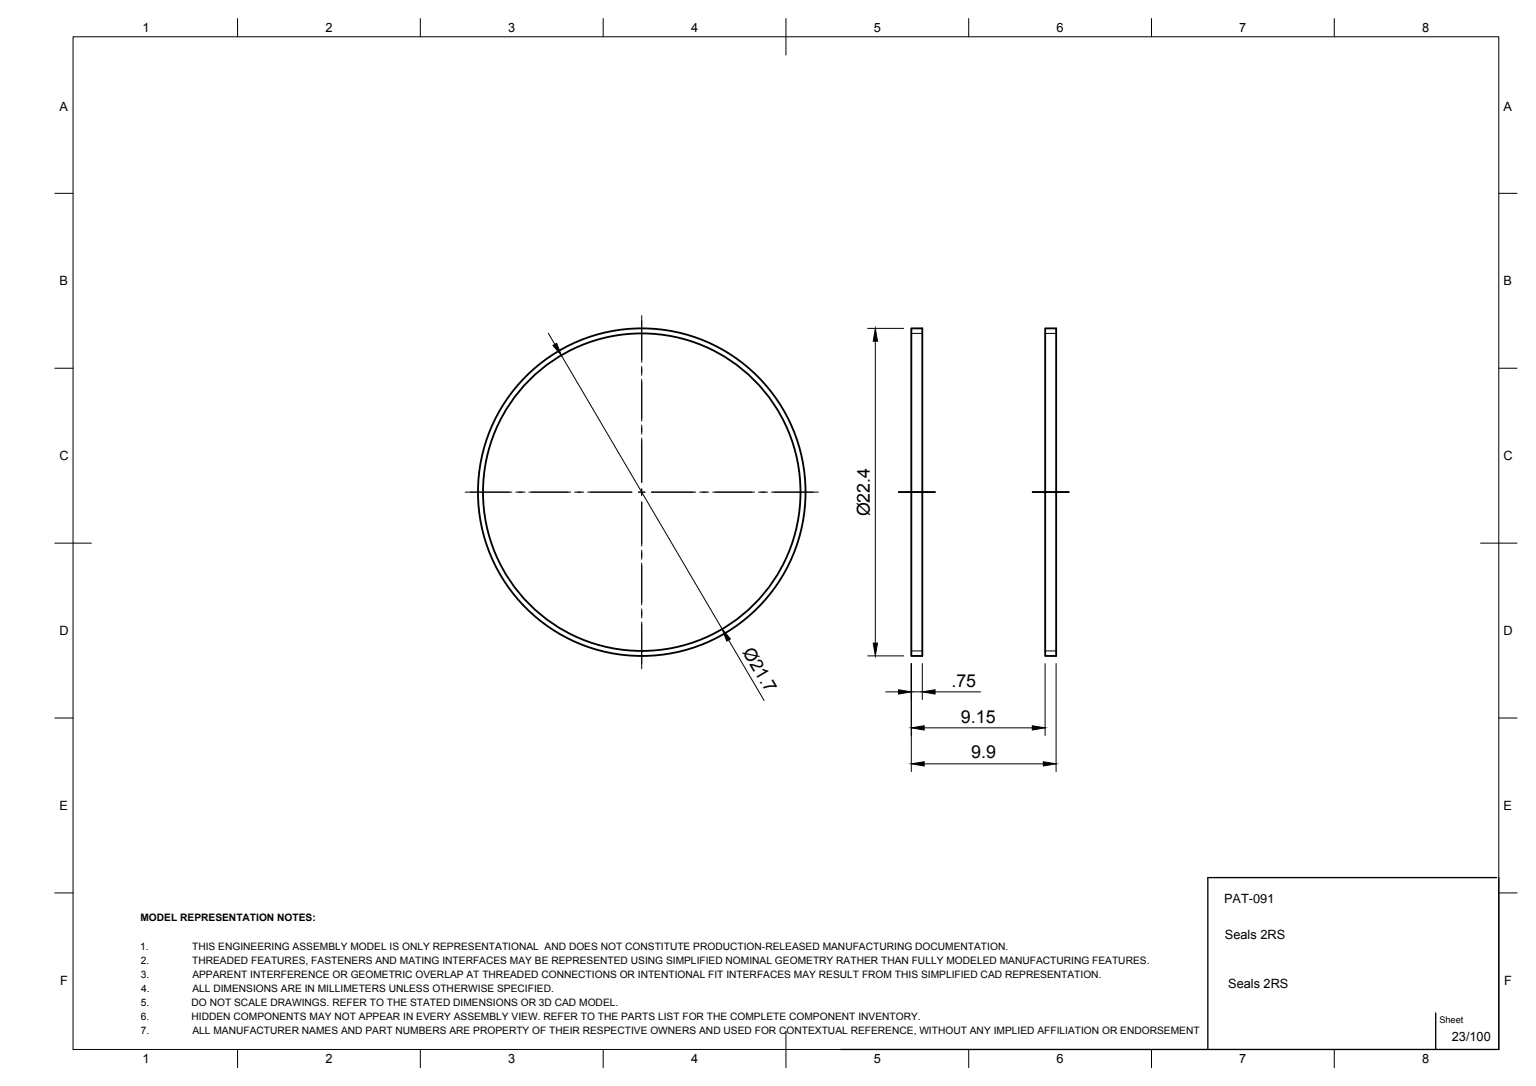
ISO-10303-21;
HEADER;
/* Generated by software containing ST-Developer
 * from STEP Tools, Inc. (www.steptools.com) 
 */

FILE_DESCRIPTION(
/* description */ ('PAT-091'),
/* implementation_level */ '2;1');

FILE_NAME(
/* name */ 'Seals 2RS.step',
/* time_stamp */ '2026-10-27T15:34:44-07:00',
/* author */ (''),
/* organization */ (''),
/* preprocessor_version */ 'ST-DEVELOPER v20.2',
/* originating_system */ 'Autodesk Translation Framework v15.17.0.0',
/* authorisation */ '');

FILE_SCHEMA (('AUTOMOTIVE_DESIGN { 1 0 10303 214 3 1 1 }'));
ENDSEC;

DATA;
#10=MECHANICAL_DESIGN_GEOMETRIC_PRESENTATION_REPRESENTATION('',(#1086,#1087),#25100);
#854=SHAPE_REPRESENTATION_RELATIONSHIP('SRR','None',#25622,#964);
#964=ADVANCED_BREP_SHAPE_REPRESENTATION('',(#1207,#1208),#25092);
#1086=STYLED_ITEM('',(#26191),#1207);
#1087=STYLED_ITEM('',(#26191),#1208);
#1207=MANIFOLD_SOLID_BREP('Body1',#13366);
#1208=MANIFOLD_SOLID_BREP('Body2',#13367);
#1621=FACE_BOUND('',#4065,.T.);
#1622=FACE_BOUND('',#4068,.T.);
#1623=FACE_BOUND('',#4071,.T.);
#1624=FACE_BOUND('',#4074,.T.);
#2042=PLANE('',#16288);
#2043=PLANE('',#16293);
#2044=PLANE('',#16296);
#2045=PLANE('',#16301);
#2840=FACE_OUTER_BOUND('',#4064,.T.);
#2841=FACE_OUTER_BOUND('',#4066,.T.);
#2842=FACE_OUTER_BOUND('',#4067,.T.);
#2843=FACE_OUTER_BOUND('',#4069,.T.);
#2844=FACE_OUTER_BOUND('',#4070,.T.);
#2845=FACE_OUTER_BOUND('',#4072,.T.);
#2846=FACE_OUTER_BOUND('',#4073,.T.);
#2847=FACE_OUTER_BOUND('',#4075,.T.);
#4064=EDGE_LOOP('',(#11954));
#4065=EDGE_LOOP('',(#11955));
#4066=EDGE_LOOP('',(#11956,#11957,#11958,#11959));
#4067=EDGE_LOOP('',(#11960));
#4068=EDGE_LOOP('',(#11961));
#4069=EDGE_LOOP('',(#11962,#11963,#11964,#11965));
#4070=EDGE_LOOP('',(#11966));
#4071=EDGE_LOOP('',(#11967));
#4072=EDGE_LOOP('',(#11968,#11969,#11970,#11971));
#4073=EDGE_LOOP('',(#11972));
#4074=EDGE_LOOP('',(#11973));
#4075=EDGE_LOOP('',(#11974,#11975,#11976,#11977));
#4844=LINE('',#24627,#5584);
#4845=LINE('',#24632,#5585);
#4846=LINE('',#24641,#5586);
#4847=LINE('',#24646,#5587);
#5584=VECTOR('',#20604,1.119765);
#5585=VECTOR('',#20611,1.085235);
#5586=VECTOR('',#20622,1.119765);
#5587=VECTOR('',#20629,1.085235);
#6343=CIRCLE('',#16289,1.119765);
#6344=CIRCLE('',#16290,1.085235);
#6345=CIRCLE('',#16292,1.119765);
#6346=CIRCLE('',#16294,1.085235);
#6347=CIRCLE('',#16297,1.119765);
#6348=CIRCLE('',#16298,1.085235);
#6349=CIRCLE('',#16300,1.119765);
#6350=CIRCLE('',#16302,1.085235);
#7381=VERTEX_POINT('',#24620);
#7382=VERTEX_POINT('',#24622);
#7383=VERTEX_POINT('',#24625);
#7384=VERTEX_POINT('',#24629);
#7385=VERTEX_POINT('',#24634);
#7386=VERTEX_POINT('',#24636);
#7387=VERTEX_POINT('',#24639);
#7388=VERTEX_POINT('',#24643);
#8912=EDGE_CURVE('',#7381,#7381,#6343,.T.);
#8913=EDGE_CURVE('',#7382,#7382,#6344,.T.);
#8914=EDGE_CURVE('',#7383,#7383,#6345,.T.);
#8915=EDGE_CURVE('',#7383,#7381,#4844,.T.);
#8916=EDGE_CURVE('',#7384,#7384,#6346,.T.);
#8917=EDGE_CURVE('',#7384,#7382,#4845,.T.);
#8918=EDGE_CURVE('',#7385,#7385,#6347,.T.);
#8919=EDGE_CURVE('',#7386,#7386,#6348,.T.);
#8920=EDGE_CURVE('',#7387,#7387,#6349,.T.);
#8921=EDGE_CURVE('',#7387,#7385,#4846,.T.);
#8922=EDGE_CURVE('',#7388,#7388,#6350,.T.);
#8923=EDGE_CURVE('',#7388,#7386,#4847,.T.);
#11954=ORIENTED_EDGE('',*,*,#8912,.F.);
#11955=ORIENTED_EDGE('',*,*,#8913,.T.);
#11956=ORIENTED_EDGE('',*,*,#8914,.F.);
#11957=ORIENTED_EDGE('',*,*,#8915,.T.);
#11958=ORIENTED_EDGE('',*,*,#8912,.T.);
#11959=ORIENTED_EDGE('',*,*,#8915,.F.);
#11960=ORIENTED_EDGE('',*,*,#8914,.T.);
#11961=ORIENTED_EDGE('',*,*,#8916,.F.);
#11962=ORIENTED_EDGE('',*,*,#8916,.T.);
#11963=ORIENTED_EDGE('',*,*,#8917,.T.);
#11964=ORIENTED_EDGE('',*,*,#8913,.F.);
#11965=ORIENTED_EDGE('',*,*,#8917,.F.);
#11966=ORIENTED_EDGE('',*,*,#8918,.F.);
#11967=ORIENTED_EDGE('',*,*,#8919,.T.);
#11968=ORIENTED_EDGE('',*,*,#8920,.F.);
#11969=ORIENTED_EDGE('',*,*,#8921,.T.);
#11970=ORIENTED_EDGE('',*,*,#8918,.T.);
#11971=ORIENTED_EDGE('',*,*,#8921,.F.);
#11972=ORIENTED_EDGE('',*,*,#8920,.T.);
#11973=ORIENTED_EDGE('',*,*,#8922,.F.);
#11974=ORIENTED_EDGE('',*,*,#8922,.T.);
#11975=ORIENTED_EDGE('',*,*,#8923,.T.);
#11976=ORIENTED_EDGE('',*,*,#8919,.F.);
#11977=ORIENTED_EDGE('',*,*,#8923,.F.);
#12410=CYLINDRICAL_SURFACE('',#16291,1.119765);
#12411=CYLINDRICAL_SURFACE('',#16295,1.085235);
#12412=CYLINDRICAL_SURFACE('',#16299,1.119765);
#12413=CYLINDRICAL_SURFACE('',#16303,1.085235);
#13207=ADVANCED_FACE('',(#2840,#1621),#2042,.T.);
#13208=ADVANCED_FACE('',(#2841),#12410,.T.);
#13209=ADVANCED_FACE('',(#2842,#1622),#2043,.T.);
#13210=ADVANCED_FACE('',(#2843),#12411,.F.);
#13211=ADVANCED_FACE('',(#2844,#1623),#2044,.T.);
#13212=ADVANCED_FACE('',(#2845),#12412,.T.);
#13213=ADVANCED_FACE('',(#2846,#1624),#2045,.T.);
#13214=ADVANCED_FACE('',(#2847),#12413,.F.);
#13366=CLOSED_SHELL('',(#13207,#13208,#13209,#13210));
#13367=CLOSED_SHELL('',(#13211,#13212,#13213,#13214));
#16287=AXIS2_PLACEMENT_3D('',#24618,#20592,#20593);
#16288=AXIS2_PLACEMENT_3D('',#24619,#20594,#20595);
#16289=AXIS2_PLACEMENT_3D('',#24621,#20596,#20597);
#16290=AXIS2_PLACEMENT_3D('',#24623,#20598,#20599);
#16291=AXIS2_PLACEMENT_3D('',#24624,#20600,#20601);
#16292=AXIS2_PLACEMENT_3D('',#24626,#20602,#20603);
#16293=AXIS2_PLACEMENT_3D('',#24628,#20605,#20606);
#16294=AXIS2_PLACEMENT_3D('',#24630,#20607,#20608);
#16295=AXIS2_PLACEMENT_3D('',#24631,#20609,#20610);
#16296=AXIS2_PLACEMENT_3D('',#24633,#20612,#20613);
#16297=AXIS2_PLACEMENT_3D('',#24635,#20614,#20615);
#16298=AXIS2_PLACEMENT_3D('',#24637,#20616,#20617);
#16299=AXIS2_PLACEMENT_3D('',#24638,#20618,#20619);
#16300=AXIS2_PLACEMENT_3D('',#24640,#20620,#20621);
#16301=AXIS2_PLACEMENT_3D('',#24642,#20623,#20624);
#16302=AXIS2_PLACEMENT_3D('',#24644,#20625,#20626);
#16303=AXIS2_PLACEMENT_3D('',#24645,#20627,#20628);
#20592=DIRECTION('axis',(0.,0.,1.));
#20593=DIRECTION('refdir',(1.,0.,0.));
#20594=DIRECTION('center_axis',(0.,1.,0.));
#20595=DIRECTION('ref_axis',(0.,0.,1.));
#20596=DIRECTION('center_axis',(0.,-1.,0.));
#20597=DIRECTION('ref_axis',(1.,0.,0.));
#20598=DIRECTION('center_axis',(0.,-1.,0.));
#20599=DIRECTION('ref_axis',(1.,0.,0.));
#20600=DIRECTION('center_axis',(0.,-1.,0.));
#20601=DIRECTION('ref_axis',(1.,0.,0.));
#20602=DIRECTION('center_axis',(0.,-1.,0.));
#20603=DIRECTION('ref_axis',(1.,0.,0.));
#20604=DIRECTION('',(0.,1.,0.));
#20605=DIRECTION('center_axis',(0.,-1.,0.));
#20606=DIRECTION('ref_axis',(0.,0.,-1.));
#20607=DIRECTION('center_axis',(0.,-1.,0.));
#20608=DIRECTION('ref_axis',(1.,0.,0.));
#20609=DIRECTION('center_axis',(0.,-1.,0.));
#20610=DIRECTION('ref_axis',(1.,0.,0.));
#20611=DIRECTION('',(0.,1.,0.));
#20612=DIRECTION('center_axis',(0.,1.,0.));
#20613=DIRECTION('ref_axis',(0.,0.,1.));
#20614=DIRECTION('center_axis',(0.,-1.,0.));
#20615=DIRECTION('ref_axis',(1.,0.,0.));
#20616=DIRECTION('center_axis',(0.,-1.,0.));
#20617=DIRECTION('ref_axis',(1.,0.,0.));
#20618=DIRECTION('center_axis',(0.,-1.,0.));
#20619=DIRECTION('ref_axis',(1.,0.,0.));
#20620=DIRECTION('center_axis',(0.,-1.,0.));
#20621=DIRECTION('ref_axis',(1.,0.,0.));
#20622=DIRECTION('',(0.,1.,0.));
#20623=DIRECTION('center_axis',(0.,-1.,0.));
#20624=DIRECTION('ref_axis',(0.,0.,-1.));
#20625=DIRECTION('center_axis',(0.,-1.,0.));
#20626=DIRECTION('ref_axis',(1.,0.,0.));
#20627=DIRECTION('center_axis',(0.,-1.,0.));
#20628=DIRECTION('ref_axis',(1.,0.,0.));
#20629=DIRECTION('',(0.,1.,0.));
#24618=CARTESIAN_POINT('',(0.,0.,0.));
#24619=CARTESIAN_POINT('Origin',(1.119765,0.495,0.));
#24620=CARTESIAN_POINT('',(-1.119765,0.495,-1.37131662304724E-16));
#24621=CARTESIAN_POINT('Origin',(0.,0.495,0.));
#24622=CARTESIAN_POINT('',(-1.085235,0.495,-1.32902956907268E-16));
#24623=CARTESIAN_POINT('Origin',(0.,0.495,0.));
#24624=CARTESIAN_POINT('Origin',(0.,0.4575,0.));
#24625=CARTESIAN_POINT('',(-1.119765,0.42,-1.37131662304724E-16));
#24626=CARTESIAN_POINT('Origin',(0.,0.42,0.));
#24627=CARTESIAN_POINT('',(-1.119765,0.4575,-1.37131662304724E-16));
#24628=CARTESIAN_POINT('Origin',(1.085235,0.42,0.));
#24629=CARTESIAN_POINT('',(-1.085235,0.42,-1.32902956907268E-16));
#24630=CARTESIAN_POINT('Origin',(0.,0.42,0.));
#24631=CARTESIAN_POINT('Origin',(0.,0.4575,0.));
#24632=CARTESIAN_POINT('',(-1.085235,0.4575,-1.32902956907268E-16));
#24633=CARTESIAN_POINT('Origin',(1.119765,-0.42,0.));
#24634=CARTESIAN_POINT('',(-1.119765,-0.42,-1.37131662304724E-16));
#24635=CARTESIAN_POINT('Origin',(0.,-0.42,0.));
#24636=CARTESIAN_POINT('',(-1.085235,-0.42,-1.32902956907268E-16));
#24637=CARTESIAN_POINT('Origin',(0.,-0.42,0.));
#24638=CARTESIAN_POINT('Origin',(0.,-0.4575,0.));
#24639=CARTESIAN_POINT('',(-1.119765,-0.495,-1.37131662304724E-16));
#24640=CARTESIAN_POINT('Origin',(0.,-0.495,0.));
#24641=CARTESIAN_POINT('',(-1.119765,-0.4575,-1.37131662304724E-16));
#24642=CARTESIAN_POINT('Origin',(1.085235,-0.495,0.));
#24643=CARTESIAN_POINT('',(-1.085235,-0.495,-1.32902956907268E-16));
#24644=CARTESIAN_POINT('Origin',(0.,-0.495,0.));
#24645=CARTESIAN_POINT('Origin',(0.,-0.4575,0.));
#24646=CARTESIAN_POINT('',(-1.085235,-0.4575,-1.32902956907268E-16));
#24971=UNCERTAINTY_MEASURE_WITH_UNIT(LENGTH_MEASURE(0.001),#25101,
'DISTANCE_ACCURACY_VALUE',
'Maximum model space distance between geometric entities at asserted c
onnectivities');
#24979=UNCERTAINTY_MEASURE_WITH_UNIT(LENGTH_MEASURE(0.001),#25101,
'DISTANCE_ACCURACY_VALUE',
'Maximum model space distance between geometric entities at asserted c
onnectivities');
#25092=(
GEOMETRIC_REPRESENTATION_CONTEXT(3)
GLOBAL_UNCERTAINTY_ASSIGNED_CONTEXT((#24971))
GLOBAL_UNIT_ASSIGNED_CONTEXT((#25101,#25103,#25104))
REPRESENTATION_CONTEXT('','3D')
);
#25100=(
GEOMETRIC_REPRESENTATION_CONTEXT(3)
GLOBAL_UNCERTAINTY_ASSIGNED_CONTEXT((#24979))
GLOBAL_UNIT_ASSIGNED_CONTEXT((#25101,#25103,#25104))
REPRESENTATION_CONTEXT('','3D')
);
#25101=(
LENGTH_UNIT()
NAMED_UNIT(*)
SI_UNIT(.CENTI.,.METRE.)
);
#25103=(
NAMED_UNIT(*)
PLANE_ANGLE_UNIT()
SI_UNIT($,.RADIAN.)
);
#25104=(
NAMED_UNIT(*)
SI_UNIT($,.STERADIAN.)
SOLID_ANGLE_UNIT()
);
#25217=SHAPE_DEFINITION_REPRESENTATION(#25411,#25622);
#25411=PRODUCT_DEFINITION_SHAPE('',$,#25743);
#25622=SHAPE_REPRESENTATION('',(#16287),#25092);
#25630=PRODUCT_DEFINITION_CONTEXT('part definition',#25992,'design');
#25743=PRODUCT_DEFINITION('Seals 2RS','Seals 2RS',#25863,#25630);
#25863=PRODUCT_DEFINITION_FORMATION('',$,#26106);
#25992=APPLICATION_CONTEXT(
'Core Data for Automotive Mechanical Design Process');
#25993=PRODUCT_CONTEXT('part definition',#25992,'mechanical');
#26106=PRODUCT('Seals 2RS','Seals 2RS','Seals 2RS',(#25993));
#26185=COLOUR_RGB('Grey',0.48,0.52,0.57);
#26186=FILL_AREA_STYLE_COLOUR('',#26185);
#26187=FILL_AREA_STYLE('',(#26186));
#26188=SURFACE_STYLE_FILL_AREA(#26187);
#26189=SURFACE_SIDE_STYLE('',(#26188));
#26190=SURFACE_STYLE_USAGE(.BOTH.,#26189);
#26191=PRESENTATION_STYLE_ASSIGNMENT((#26190));
ENDSEC;
END-ISO-10303-21;
